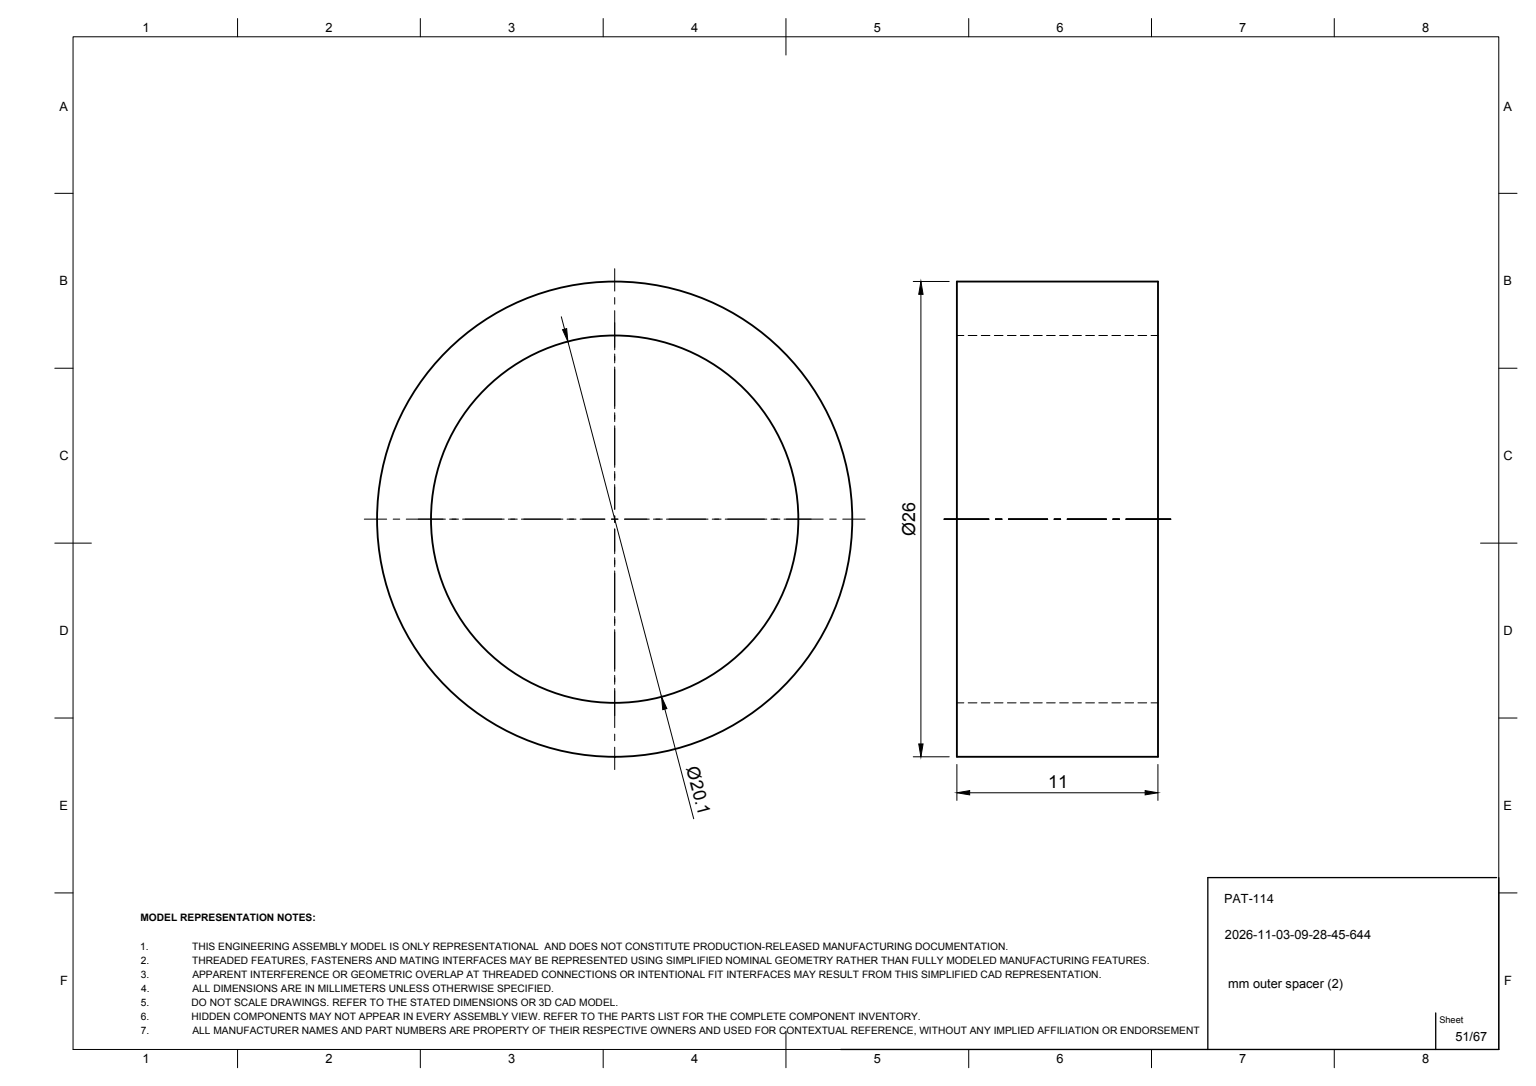
ISO-10303-21;
HEADER;
/* Generated by software containing ST-Developer
 * from STEP Tools, Inc. (www.steptools.com) 
 */

FILE_DESCRIPTION(
/* description */ ('Two-stage gear reducer in split housing'),
/* implementation_level */ '2;1');

FILE_NAME(
/* name */ 'mm outer spacer (2).step',
/* time_stamp */ '2026-10-28T03:22:31-07:00',
/* author */ (''),
/* organization */ (''),
/* preprocessor_version */ 'ST-DEVELOPER v20.2',
/* originating_system */ 'Autodesk Translation Framework v15.17.0.0',
/* authorisation */ '');

FILE_SCHEMA (('AUTOMOTIVE_DESIGN { 1 0 10303 214 3 1 1 }'));
ENDSEC;

DATA;
#10=MECHANICAL_DESIGN_GEOMETRIC_PRESENTATION_REPRESENTATION('',(#1289),#73366);
#1162=SHAPE_REPRESENTATION_RELATIONSHIP('SRR','None',#73653,#1218);
#1218=ADVANCED_BREP_SHAPE_REPRESENTATION('',(#1358),#73349);
#1289=STYLED_ITEM('',(#73974),#1358);
#1358=MANIFOLD_SOLID_BREP('Body1',#16179);
#1568=FACE_BOUND('',#3689,.T.);
#1569=FACE_BOUND('',#3691,.T.);
#1878=PLANE('',#18006);
#1879=PLANE('',#18007);
#2579=FACE_OUTER_BOUND('',#3686,.T.);
#2580=FACE_OUTER_BOUND('',#3687,.T.);
#2581=FACE_OUTER_BOUND('',#3688,.T.);
#2582=FACE_OUTER_BOUND('',#3690,.T.);
#3686=EDGE_LOOP('',(#13107,#13108,#13109,#13110));
#3687=EDGE_LOOP('',(#13111,#13112,#13113,#13114));
#3688=EDGE_LOOP('',(#13115));
#3689=EDGE_LOOP('',(#13116));
#3690=EDGE_LOOP('',(#13117));
#3691=EDGE_LOOP('',(#13118));
#4694=LINE('',#37591,#5718);
#4695=LINE('',#37597,#5719);
#5718=VECTOR('',#21476,1.005);
#5719=VECTOR('',#21483,1.3);
#6638=CIRCLE('',#18001,1.005);
#6639=CIRCLE('',#18002,1.005);
#6640=CIRCLE('',#18004,1.3);
#6641=CIRCLE('',#18005,1.3);
#7707=VERTEX_POINT('',#37588);
#7708=VERTEX_POINT('',#37590);
#7709=VERTEX_POINT('',#37594);
#7710=VERTEX_POINT('',#37596);
#9607=EDGE_CURVE('',#7707,#7707,#6638,.T.);
#9608=EDGE_CURVE('',#7707,#7708,#4694,.T.);
#9609=EDGE_CURVE('',#7708,#7708,#6639,.T.);
#9610=EDGE_CURVE('',#7709,#7709,#6640,.T.);
#9611=EDGE_CURVE('',#7709,#7710,#4695,.T.);
#9612=EDGE_CURVE('',#7710,#7710,#6641,.T.);
#13107=ORIENTED_EDGE('',*,*,#9607,.F.);
#13108=ORIENTED_EDGE('',*,*,#9608,.T.);
#13109=ORIENTED_EDGE('',*,*,#9609,.T.);
#13110=ORIENTED_EDGE('',*,*,#9608,.F.);
#13111=ORIENTED_EDGE('',*,*,#9610,.F.);
#13112=ORIENTED_EDGE('',*,*,#9611,.T.);
#13113=ORIENTED_EDGE('',*,*,#9612,.T.);
#13114=ORIENTED_EDGE('',*,*,#9611,.F.);
#13115=ORIENTED_EDGE('',*,*,#9610,.T.);
#13116=ORIENTED_EDGE('',*,*,#9607,.T.);
#13117=ORIENTED_EDGE('',*,*,#9612,.F.);
#13118=ORIENTED_EDGE('',*,*,#9609,.F.);
#15119=CYLINDRICAL_SURFACE('',#18000,1.005);
#15120=CYLINDRICAL_SURFACE('',#18003,1.3);
#15786=ADVANCED_FACE('',(#2579),#15119,.F.);
#15787=ADVANCED_FACE('',(#2580),#15120,.T.);
#15788=ADVANCED_FACE('',(#2581,#1568),#1878,.T.);
#15789=ADVANCED_FACE('',(#2582,#1569),#1879,.F.);
#16179=CLOSED_SHELL('',(#15786,#15787,#15788,#15789));
#17999=AXIS2_PLACEMENT_3D('',#37586,#21470,#21471);
#18000=AXIS2_PLACEMENT_3D('',#37587,#21472,#21473);
#18001=AXIS2_PLACEMENT_3D('',#37589,#21474,#21475);
#18002=AXIS2_PLACEMENT_3D('',#37592,#21477,#21478);
#18003=AXIS2_PLACEMENT_3D('',#37593,#21479,#21480);
#18004=AXIS2_PLACEMENT_3D('',#37595,#21481,#21482);
#18005=AXIS2_PLACEMENT_3D('',#37598,#21484,#21485);
#18006=AXIS2_PLACEMENT_3D('',#37599,#21486,#21487);
#18007=AXIS2_PLACEMENT_3D('',#37600,#21488,#21489);
#21470=DIRECTION('axis',(0.,0.,1.));
#21471=DIRECTION('refdir',(1.,0.,0.));
#21472=DIRECTION('center_axis',(0.,1.,0.));
#21473=DIRECTION('ref_axis',(1.,0.,0.));
#21474=DIRECTION('center_axis',(0.,-1.,0.));
#21475=DIRECTION('ref_axis',(1.,0.,0.));
#21476=DIRECTION('',(0.,-1.,0.));
#21477=DIRECTION('center_axis',(0.,-1.,0.));
#21478=DIRECTION('ref_axis',(1.,0.,0.));
#21479=DIRECTION('center_axis',(0.,1.,0.));
#21480=DIRECTION('ref_axis',(1.,0.,0.));
#21481=DIRECTION('center_axis',(0.,1.,0.));
#21482=DIRECTION('ref_axis',(1.,0.,0.));
#21483=DIRECTION('',(0.,-1.,0.));
#21484=DIRECTION('center_axis',(0.,1.,0.));
#21485=DIRECTION('ref_axis',(1.,0.,0.));
#21486=DIRECTION('center_axis',(0.,1.,0.));
#21487=DIRECTION('ref_axis',(1.,0.,0.));
#21488=DIRECTION('center_axis',(0.,1.,0.));
#21489=DIRECTION('ref_axis',(1.,0.,0.));
#37586=CARTESIAN_POINT('',(0.,0.,0.));
#37587=CARTESIAN_POINT('Origin',(6.,-7.8,10.));
#37588=CARTESIAN_POINT('',(4.995,-6.7,10.));
#37589=CARTESIAN_POINT('Origin',(6.,-6.7,10.));
#37590=CARTESIAN_POINT('',(4.995,-7.8,10.));
#37591=CARTESIAN_POINT('',(4.995,-7.8,10.));
#37592=CARTESIAN_POINT('Origin',(6.,-7.8,10.));
#37593=CARTESIAN_POINT('Origin',(6.,-7.8,10.));
#37594=CARTESIAN_POINT('',(4.7,-6.7,10.));
#37595=CARTESIAN_POINT('Origin',(6.,-6.7,10.));
#37596=CARTESIAN_POINT('',(4.7,-7.8,10.));
#37597=CARTESIAN_POINT('',(4.7,-7.8,10.));
#37598=CARTESIAN_POINT('Origin',(6.,-7.8,10.));
#37599=CARTESIAN_POINT('Origin',(6.,-6.7,10.));
#37600=CARTESIAN_POINT('Origin',(6.,-7.8,10.));
#73285=UNCERTAINTY_MEASURE_WITH_UNIT(LENGTH_MEASURE(0.001),#73367,
'DISTANCE_ACCURACY_VALUE',
'Maximum model space distance between geometric entities at asserted c
onnectivities');
#73302=UNCERTAINTY_MEASURE_WITH_UNIT(LENGTH_MEASURE(0.001),#73367,
'DISTANCE_ACCURACY_VALUE',
'Maximum model space distance between geometric entities at asserted c
onnectivities');
#73349=(
GEOMETRIC_REPRESENTATION_CONTEXT(3)
GLOBAL_UNCERTAINTY_ASSIGNED_CONTEXT((#73285))
GLOBAL_UNIT_ASSIGNED_CONTEXT((#73367,#73369,#73370))
REPRESENTATION_CONTEXT('','3D')
);
#73366=(
GEOMETRIC_REPRESENTATION_CONTEXT(3)
GLOBAL_UNCERTAINTY_ASSIGNED_CONTEXT((#73302))
GLOBAL_UNIT_ASSIGNED_CONTEXT((#73367,#73369,#73370))
REPRESENTATION_CONTEXT('','3D')
);
#73367=(
LENGTH_UNIT()
NAMED_UNIT(*)
SI_UNIT(.CENTI.,.METRE.)
);
#73369=(
NAMED_UNIT(*)
PLANE_ANGLE_UNIT()
SI_UNIT($,.RADIAN.)
);
#73370=(
NAMED_UNIT(*)
SI_UNIT($,.STERADIAN.)
SOLID_ANGLE_UNIT()
);
#73417=SHAPE_DEFINITION_REPRESENTATION(#73550,#73653);
#73550=PRODUCT_DEFINITION_SHAPE('',$,#73717);
#73653=SHAPE_REPRESENTATION('',(#17999),#73349);
#73670=PRODUCT_DEFINITION_CONTEXT('part definition',#73861,'design');
#73717=PRODUCT_DEFINITION('mm outer spacer (2)','mm outer spacer (2)',#73780,
#73670);
#73780=PRODUCT_DEFINITION_FORMATION('',$,#73909);
#73861=APPLICATION_CONTEXT(
'Core Data for Automotive Mechanical Design Process');
#73862=PRODUCT_CONTEXT('part definition',#73861,'mechanical');
#73909=PRODUCT('mm outer spacer (2)','mm outer spacer (2)',
'mm outer spacer (2)',(#73862));
#73968=COLOUR_RGB('Light Blue',0.38,0.62,0.78);
#73969=FILL_AREA_STYLE_COLOUR('',#73968);
#73970=FILL_AREA_STYLE('',(#73969));
#73971=SURFACE_STYLE_FILL_AREA(#73970);
#73972=SURFACE_SIDE_STYLE('',(#73971));
#73973=SURFACE_STYLE_USAGE(.BOTH.,#73972);
#73974=PRESENTATION_STYLE_ASSIGNMENT((#73973));
ENDSEC;
END-ISO-10303-21;
